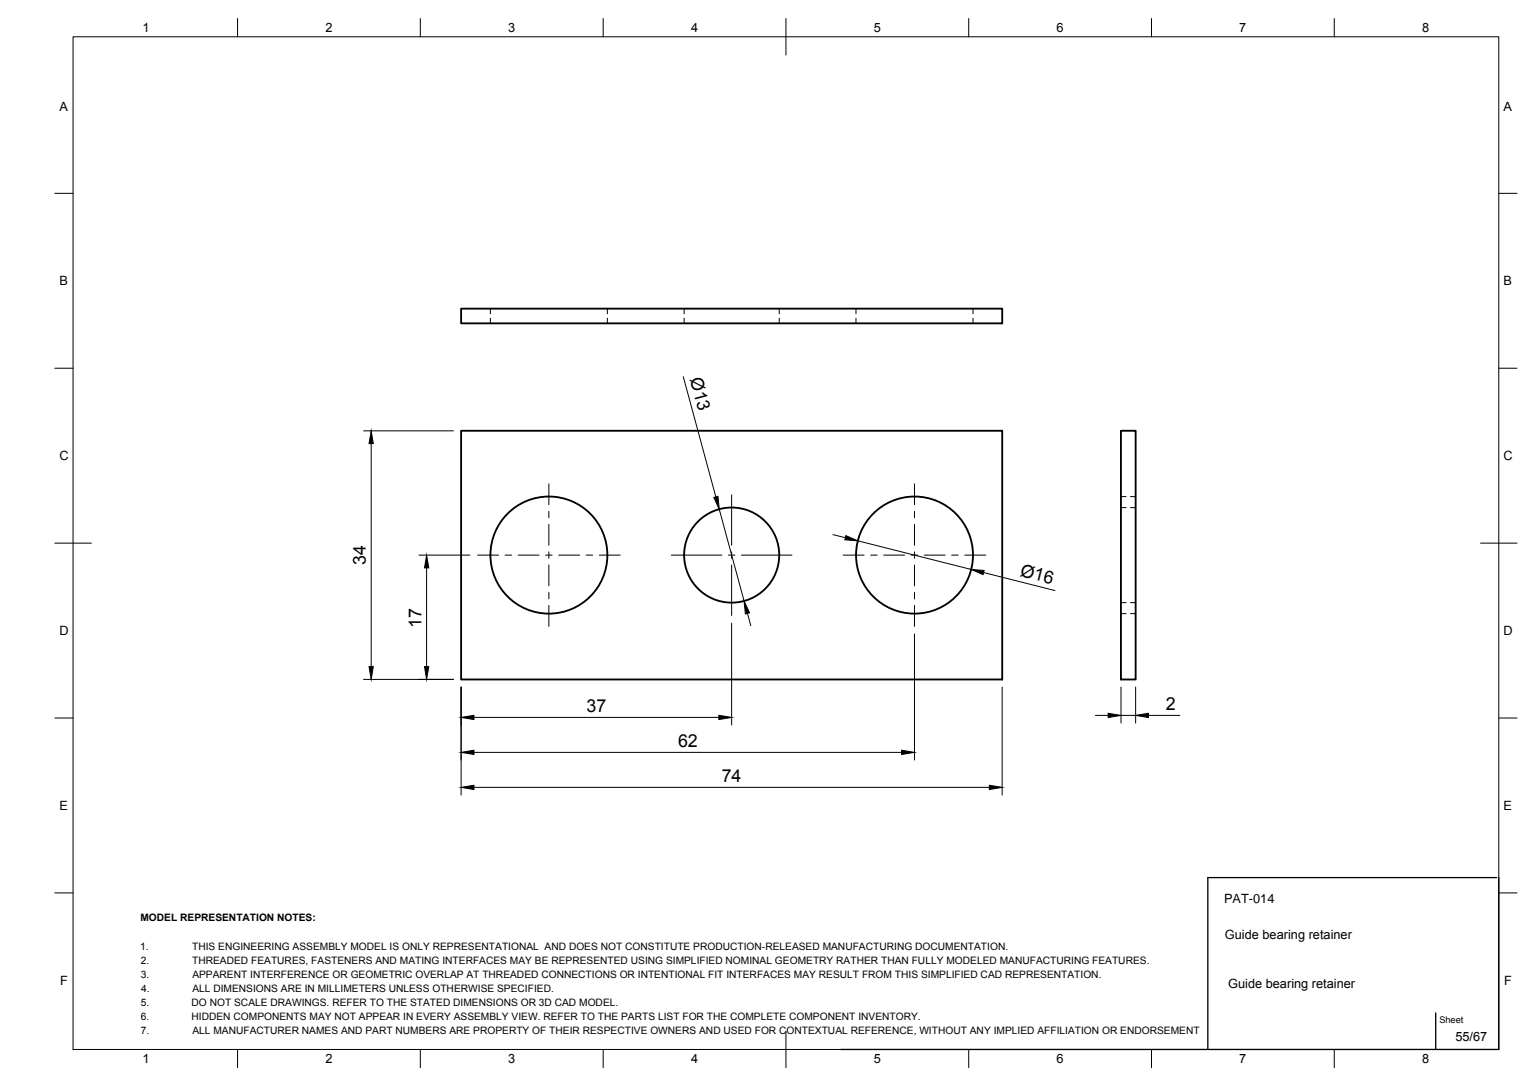
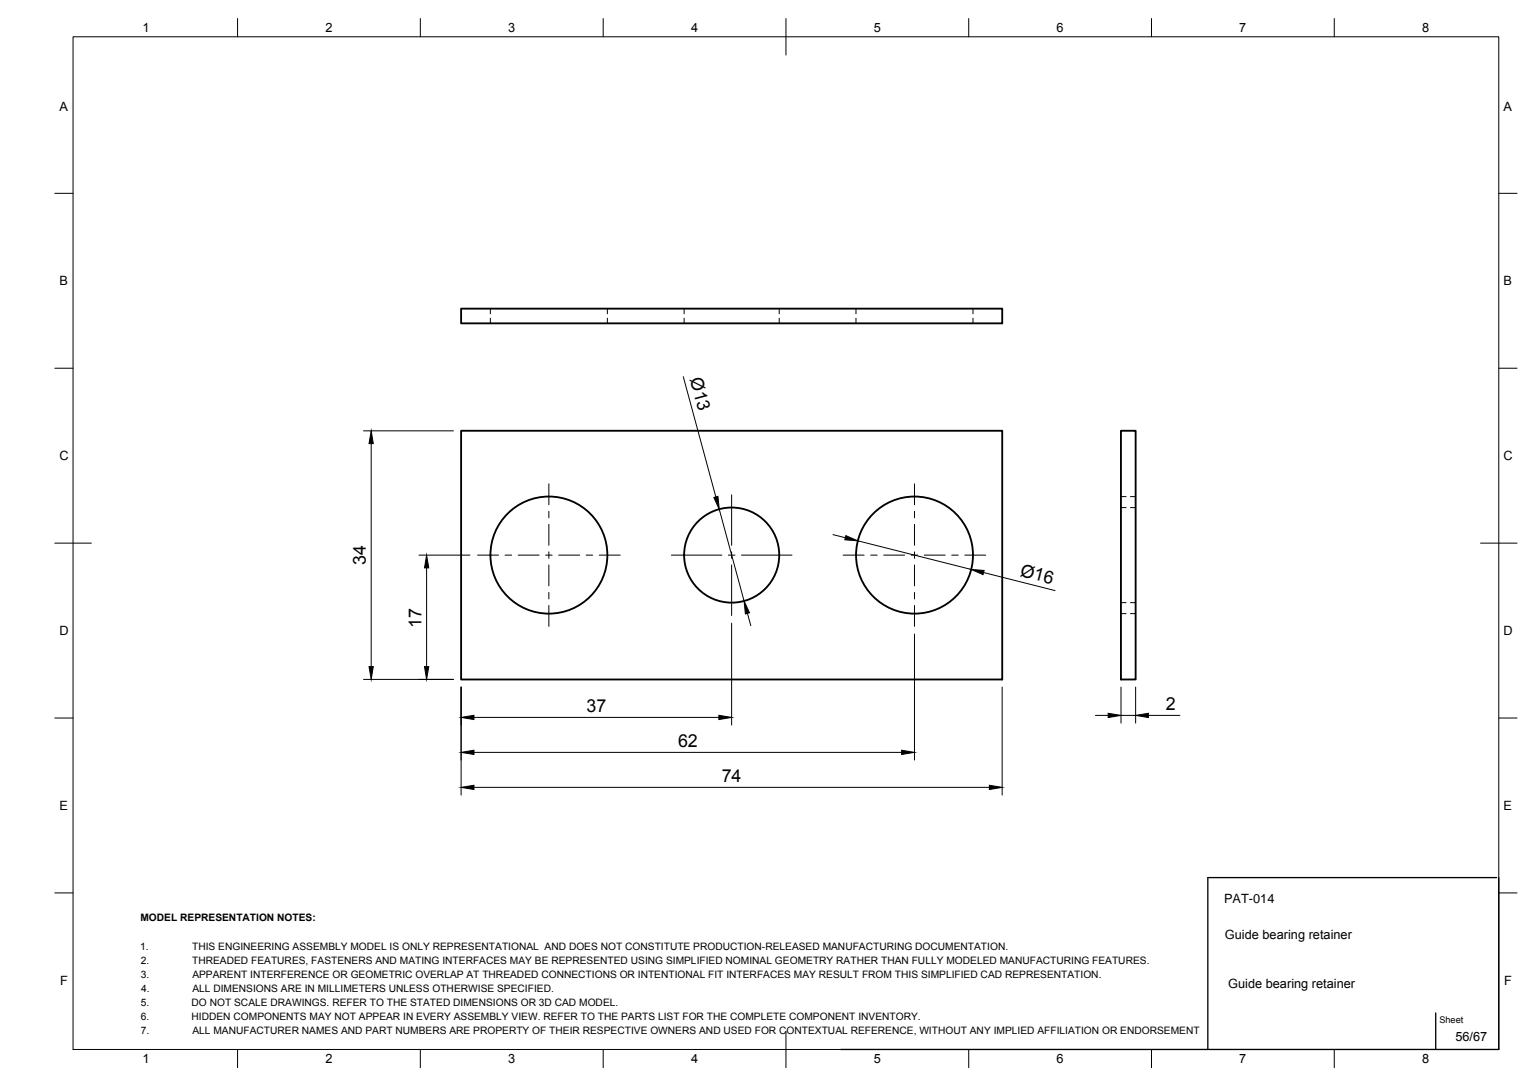
ISO-10303-21;
HEADER;
/* Generated by software containing ST-Developer
 * from STEP Tools, Inc. (www.steptools.com) 
 */

FILE_DESCRIPTION(
/* description */ ('Bin tilter linkage'),
/* implementation_level */ '2;1');

FILE_NAME(
/* name */ 'Guide bearing retainer.step',
/* time_stamp */ '2026-10-28T03:26:24-07:00',
/* author */ (''),
/* organization */ (''),
/* preprocessor_version */ 'ST-DEVELOPER v20.2',
/* originating_system */ 'Autodesk Translation Framework v15.17.0.0',
/* authorisation */ '');

FILE_SCHEMA (('AUTOMOTIVE_DESIGN { 1 0 10303 214 3 1 1 }'));
ENDSEC;

DATA;
#10=MECHANICAL_DESIGN_GEOMETRIC_PRESENTATION_REPRESENTATION('',(#961),#23728);
#741=SHAPE_REPRESENTATION_RELATIONSHIP('SRR','None',#24210,#847);
#847=ADVANCED_BREP_SHAPE_REPRESENTATION('',(#1073),#23710);
#961=STYLED_ITEM('',(#24765),#1073);
#1073=MANIFOLD_SOLID_BREP('Body1',#12493);
#1450=FACE_BOUND('',#3708,.T.);
#1451=FACE_BOUND('',#3709,.T.);
#1452=FACE_BOUND('',#3710,.T.);
#1453=FACE_BOUND('',#3712,.T.);
#1454=FACE_BOUND('',#3713,.T.);
#1455=FACE_BOUND('',#3714,.T.);
#1822=PLANE('',#15253);
#1823=PLANE('',#15254);
#1824=PLANE('',#15255);
#1825=PLANE('',#15256);
#1826=PLANE('',#15257);
#1827=PLANE('',#15258);
#2560=FACE_OUTER_BOUND('',#3700,.T.);
#2561=FACE_OUTER_BOUND('',#3701,.T.);
#2562=FACE_OUTER_BOUND('',#3702,.T.);
#2563=FACE_OUTER_BOUND('',#3703,.T.);
#2564=FACE_OUTER_BOUND('',#3704,.T.);
#2565=FACE_OUTER_BOUND('',#3705,.T.);
#2566=FACE_OUTER_BOUND('',#3706,.T.);
#2567=FACE_OUTER_BOUND('',#3707,.T.);
#2568=FACE_OUTER_BOUND('',#3711,.T.);
#3700=EDGE_LOOP('',(#10871,#10872,#10873,#10874));
#3701=EDGE_LOOP('',(#10875,#10876,#10877,#10878));
#3702=EDGE_LOOP('',(#10879,#10880,#10881,#10882));
#3703=EDGE_LOOP('',(#10883,#10884,#10885,#10886));
#3704=EDGE_LOOP('',(#10887,#10888,#10889,#10890));
#3705=EDGE_LOOP('',(#10891,#10892,#10893,#10894));
#3706=EDGE_LOOP('',(#10895,#10896,#10897,#10898));
#3707=EDGE_LOOP('',(#10899,#10900,#10901,#10902));
#3708=EDGE_LOOP('',(#10903));
#3709=EDGE_LOOP('',(#10904));
#3710=EDGE_LOOP('',(#10905));
#3711=EDGE_LOOP('',(#10906,#10907,#10908,#10909));
#3712=EDGE_LOOP('',(#10910));
#3713=EDGE_LOOP('',(#10911));
#3714=EDGE_LOOP('',(#10912));
#4407=LINE('',#23021,#5082);
#4408=LINE('',#23027,#5083);
#4409=LINE('',#23033,#5084);
#4410=LINE('',#23038,#5085);
#4411=LINE('',#23040,#5086);
#4412=LINE('',#23042,#5087);
#4413=LINE('',#23043,#5088);
#4414=LINE('',#23046,#5089);
#4415=LINE('',#23048,#5090);
#4416=LINE('',#23049,#5091);
#4417=LINE('',#23052,#5092);
#4418=LINE('',#23054,#5093);
#4419=LINE('',#23055,#5094);
#4420=LINE('',#23057,#5095);
#4421=LINE('',#23058,#5096);
#5082=VECTOR('',#19172,0.65);
#5083=VECTOR('',#19179,0.8);
#5084=VECTOR('',#19186,0.8);
#5085=VECTOR('',#19191,1.);
#5086=VECTOR('',#19192,1.);
#5087=VECTOR('',#19193,1.);
#5088=VECTOR('',#19194,1.);
#5089=VECTOR('',#19197,1.);
#5090=VECTOR('',#19198,1.);
#5091=VECTOR('',#19199,1.);
#5092=VECTOR('',#19202,1.);
#5093=VECTOR('',#19203,1.);
#5094=VECTOR('',#19204,1.);
#5095=VECTOR('',#19207,1.);
#5096=VECTOR('',#19208,1.);
#5876=CIRCLE('',#15245,0.65);
#5877=CIRCLE('',#15246,0.65);
#5878=CIRCLE('',#15248,0.8);
#5879=CIRCLE('',#15249,0.8);
#5880=CIRCLE('',#15251,0.8);
#5881=CIRCLE('',#15252,0.8);
#6795=VERTEX_POINT('',#23018);
#6796=VERTEX_POINT('',#23020);
#6797=VERTEX_POINT('',#23024);
#6798=VERTEX_POINT('',#23026);
#6799=VERTEX_POINT('',#23030);
#6800=VERTEX_POINT('',#23032);
#6801=VERTEX_POINT('',#23036);
#6802=VERTEX_POINT('',#23037);
#6803=VERTEX_POINT('',#23039);
#6804=VERTEX_POINT('',#23041);
#6805=VERTEX_POINT('',#23045);
#6806=VERTEX_POINT('',#23047);
#6807=VERTEX_POINT('',#23051);
#6808=VERTEX_POINT('',#23053);
#8175=EDGE_CURVE('',#6795,#6795,#5876,.T.);
#8176=EDGE_CURVE('',#6795,#6796,#4407,.T.);
#8177=EDGE_CURVE('',#6796,#6796,#5877,.T.);
#8178=EDGE_CURVE('',#6797,#6797,#5878,.T.);
#8179=EDGE_CURVE('',#6797,#6798,#4408,.T.);
#8180=EDGE_CURVE('',#6798,#6798,#5879,.T.);
#8181=EDGE_CURVE('',#6799,#6799,#5880,.T.);
#8182=EDGE_CURVE('',#6799,#6800,#4409,.T.);
#8183=EDGE_CURVE('',#6800,#6800,#5881,.T.);
#8184=EDGE_CURVE('',#6801,#6802,#4410,.T.);
#8185=EDGE_CURVE('',#6802,#6803,#4411,.T.);
#8186=EDGE_CURVE('',#6804,#6803,#4412,.T.);
#8187=EDGE_CURVE('',#6801,#6804,#4413,.T.);
#8188=EDGE_CURVE('',#6805,#6801,#4414,.T.);
#8189=EDGE_CURVE('',#6806,#6804,#4415,.T.);
#8190=EDGE_CURVE('',#6805,#6806,#4416,.T.);
#8191=EDGE_CURVE('',#6807,#6805,#4417,.T.);
#8192=EDGE_CURVE('',#6808,#6806,#4418,.T.);
#8193=EDGE_CURVE('',#6807,#6808,#4419,.T.);
#8194=EDGE_CURVE('',#6802,#6807,#4420,.T.);
#8195=EDGE_CURVE('',#6803,#6808,#4421,.T.);
#10871=ORIENTED_EDGE('',*,*,#8175,.F.);
#10872=ORIENTED_EDGE('',*,*,#8176,.T.);
#10873=ORIENTED_EDGE('',*,*,#8177,.F.);
#10874=ORIENTED_EDGE('',*,*,#8176,.F.);
#10875=ORIENTED_EDGE('',*,*,#8178,.F.);
#10876=ORIENTED_EDGE('',*,*,#8179,.T.);
#10877=ORIENTED_EDGE('',*,*,#8180,.F.);
#10878=ORIENTED_EDGE('',*,*,#8179,.F.);
#10879=ORIENTED_EDGE('',*,*,#8181,.F.);
#10880=ORIENTED_EDGE('',*,*,#8182,.T.);
#10881=ORIENTED_EDGE('',*,*,#8183,.F.);
#10882=ORIENTED_EDGE('',*,*,#8182,.F.);
#10883=ORIENTED_EDGE('',*,*,#8184,.T.);
#10884=ORIENTED_EDGE('',*,*,#8185,.T.);
#10885=ORIENTED_EDGE('',*,*,#8186,.F.);
#10886=ORIENTED_EDGE('',*,*,#8187,.F.);
#10887=ORIENTED_EDGE('',*,*,#8188,.T.);
#10888=ORIENTED_EDGE('',*,*,#8187,.T.);
#10889=ORIENTED_EDGE('',*,*,#8189,.F.);
#10890=ORIENTED_EDGE('',*,*,#8190,.F.);
#10891=ORIENTED_EDGE('',*,*,#8191,.T.);
#10892=ORIENTED_EDGE('',*,*,#8190,.T.);
#10893=ORIENTED_EDGE('',*,*,#8192,.F.);
#10894=ORIENTED_EDGE('',*,*,#8193,.F.);
#10895=ORIENTED_EDGE('',*,*,#8194,.T.);
#10896=ORIENTED_EDGE('',*,*,#8193,.T.);
#10897=ORIENTED_EDGE('',*,*,#8195,.F.);
#10898=ORIENTED_EDGE('',*,*,#8185,.F.);
#10899=ORIENTED_EDGE('',*,*,#8195,.T.);
#10900=ORIENTED_EDGE('',*,*,#8192,.T.);
#10901=ORIENTED_EDGE('',*,*,#8189,.T.);
#10902=ORIENTED_EDGE('',*,*,#8186,.T.);
#10903=ORIENTED_EDGE('',*,*,#8177,.T.);
#10904=ORIENTED_EDGE('',*,*,#8180,.T.);
#10905=ORIENTED_EDGE('',*,*,#8183,.T.);
#10906=ORIENTED_EDGE('',*,*,#8194,.F.);
#10907=ORIENTED_EDGE('',*,*,#8184,.F.);
#10908=ORIENTED_EDGE('',*,*,#8188,.F.);
#10909=ORIENTED_EDGE('',*,*,#8191,.F.);
#10910=ORIENTED_EDGE('',*,*,#8175,.T.);
#10911=ORIENTED_EDGE('',*,*,#8178,.T.);
#10912=ORIENTED_EDGE('',*,*,#8181,.T.);
#11579=CYLINDRICAL_SURFACE('',#15244,0.65);
#11580=CYLINDRICAL_SURFACE('',#15247,0.8);
#11581=CYLINDRICAL_SURFACE('',#15250,0.8);
#12285=ADVANCED_FACE('',(#2560),#11579,.F.);
#12286=ADVANCED_FACE('',(#2561),#11580,.F.);
#12287=ADVANCED_FACE('',(#2562),#11581,.F.);
#12288=ADVANCED_FACE('',(#2563),#1822,.T.);
#12289=ADVANCED_FACE('',(#2564),#1823,.T.);
#12290=ADVANCED_FACE('',(#2565),#1824,.T.);
#12291=ADVANCED_FACE('',(#2566),#1825,.T.);
#12292=ADVANCED_FACE('',(#2567,#1450,#1451,#1452),#1826,.T.);
#12293=ADVANCED_FACE('',(#2568,#1453,#1454,#1455),#1827,.F.);
#12493=CLOSED_SHELL('',(#12285,#12286,#12287,#12288,#12289,#12290,#12291,
#12292,#12293));
#15243=AXIS2_PLACEMENT_3D('',#23016,#19166,#19167);
#15244=AXIS2_PLACEMENT_3D('',#23017,#19168,#19169);
#15245=AXIS2_PLACEMENT_3D('',#23019,#19170,#19171);
#15246=AXIS2_PLACEMENT_3D('',#23022,#19173,#19174);
#15247=AXIS2_PLACEMENT_3D('',#23023,#19175,#19176);
#15248=AXIS2_PLACEMENT_3D('',#23025,#19177,#19178);
#15249=AXIS2_PLACEMENT_3D('',#23028,#19180,#19181);
#15250=AXIS2_PLACEMENT_3D('',#23029,#19182,#19183);
#15251=AXIS2_PLACEMENT_3D('',#23031,#19184,#19185);
#15252=AXIS2_PLACEMENT_3D('',#23034,#19187,#19188);
#15253=AXIS2_PLACEMENT_3D('',#23035,#19189,#19190);
#15254=AXIS2_PLACEMENT_3D('',#23044,#19195,#19196);
#15255=AXIS2_PLACEMENT_3D('',#23050,#19200,#19201);
#15256=AXIS2_PLACEMENT_3D('',#23056,#19205,#19206);
#15257=AXIS2_PLACEMENT_3D('',#23059,#19209,#19210);
#15258=AXIS2_PLACEMENT_3D('',#23060,#19211,#19212);
#19166=DIRECTION('axis',(0.,0.,1.));
#19167=DIRECTION('refdir',(1.,0.,0.));
#19168=DIRECTION('center_axis',(1.,0.,0.));
#19169=DIRECTION('ref_axis',(0.,0.,-1.));
#19170=DIRECTION('center_axis',(1.,0.,0.));
#19171=DIRECTION('ref_axis',(0.,0.,-1.));
#19172=DIRECTION('',(1.,0.,0.));
#19173=DIRECTION('center_axis',(-1.,0.,0.));
#19174=DIRECTION('ref_axis',(0.,0.,-1.));
#19175=DIRECTION('center_axis',(1.,0.,0.));
#19176=DIRECTION('ref_axis',(0.,0.,-1.));
#19177=DIRECTION('center_axis',(1.,0.,0.));
#19178=DIRECTION('ref_axis',(0.,0.,-1.));
#19179=DIRECTION('',(1.,0.,0.));
#19180=DIRECTION('center_axis',(-1.,0.,0.));
#19181=DIRECTION('ref_axis',(0.,0.,-1.));
#19182=DIRECTION('center_axis',(1.,0.,0.));
#19183=DIRECTION('ref_axis',(0.,0.,-1.));
#19184=DIRECTION('center_axis',(1.,0.,0.));
#19185=DIRECTION('ref_axis',(0.,0.,-1.));
#19186=DIRECTION('',(1.,0.,0.));
#19187=DIRECTION('center_axis',(-1.,0.,0.));
#19188=DIRECTION('ref_axis',(0.,0.,-1.));
#19189=DIRECTION('center_axis',(0.,0.,1.));
#19190=DIRECTION('ref_axis',(0.,-1.,0.));
#19191=DIRECTION('',(0.,-1.,0.));
#19192=DIRECTION('',(1.,0.,0.));
#19193=DIRECTION('',(0.,-1.,0.));
#19194=DIRECTION('',(1.,0.,0.));
#19195=DIRECTION('center_axis',(0.,1.,0.));
#19196=DIRECTION('ref_axis',(0.,0.,1.));
#19197=DIRECTION('',(0.,0.,1.));
#19198=DIRECTION('',(0.,0.,1.));
#19199=DIRECTION('',(1.,0.,0.));
#19200=DIRECTION('center_axis',(0.,0.,-1.));
#19201=DIRECTION('ref_axis',(0.,1.,0.));
#19202=DIRECTION('',(0.,1.,0.));
#19203=DIRECTION('',(0.,1.,0.));
#19204=DIRECTION('',(1.,0.,0.));
#19205=DIRECTION('center_axis',(0.,-1.,0.));
#19206=DIRECTION('ref_axis',(0.,0.,-1.));
#19207=DIRECTION('',(0.,0.,-1.));
#19208=DIRECTION('',(0.,0.,-1.));
#19209=DIRECTION('center_axis',(1.,0.,0.));
#19210=DIRECTION('ref_axis',(0.,0.,-1.));
#19211=DIRECTION('center_axis',(1.,0.,0.));
#19212=DIRECTION('ref_axis',(0.,0.,-1.));
#23016=CARTESIAN_POINT('',(0.,0.,0.));
#23017=CARTESIAN_POINT('Origin',(-6.,-4.5,8.));
#23018=CARTESIAN_POINT('',(-5.9,-4.5,8.65));
#23019=CARTESIAN_POINT('Origin',(-5.9,-4.5,8.));
#23020=CARTESIAN_POINT('',(-5.7,-4.5,8.65));
#23021=CARTESIAN_POINT('',(-6.,-4.5,8.65));
#23022=CARTESIAN_POINT('Origin',(-5.7,-4.5,8.));
#23023=CARTESIAN_POINT('Origin',(-6.,-7.,8.));
#23024=CARTESIAN_POINT('',(-5.9,-7.,8.8));
#23025=CARTESIAN_POINT('Origin',(-5.9,-7.,8.));
#23026=CARTESIAN_POINT('',(-5.7,-7.,8.8));
#23027=CARTESIAN_POINT('',(-6.,-7.,8.8));
#23028=CARTESIAN_POINT('Origin',(-5.7,-7.,8.));
#23029=CARTESIAN_POINT('Origin',(-6.,-2.,8.));
#23030=CARTESIAN_POINT('',(-5.9,-2.,8.8));
#23031=CARTESIAN_POINT('Origin',(-5.9,-2.,8.));
#23032=CARTESIAN_POINT('',(-5.7,-2.,8.8));
#23033=CARTESIAN_POINT('',(-6.,-2.,8.8));
#23034=CARTESIAN_POINT('Origin',(-5.7,-2.,8.));
#23035=CARTESIAN_POINT('Origin',(-5.9,-0.8,9.7));
#23036=CARTESIAN_POINT('',(-5.9,-0.8,9.7));
#23037=CARTESIAN_POINT('',(-5.9,-8.2,9.7));
#23038=CARTESIAN_POINT('',(-5.9,-0.8,9.7));
#23039=CARTESIAN_POINT('',(-5.7,-8.2,9.7));
#23040=CARTESIAN_POINT('',(-5.9,-8.2,9.7));
#23041=CARTESIAN_POINT('',(-5.7,-0.8,9.7));
#23042=CARTESIAN_POINT('',(-5.7,-0.8,9.7));
#23043=CARTESIAN_POINT('',(-5.9,-0.8,9.7));
#23044=CARTESIAN_POINT('Origin',(-5.9,-0.8,6.3));
#23045=CARTESIAN_POINT('',(-5.9,-0.8,6.3));
#23046=CARTESIAN_POINT('',(-5.9,-0.8,6.3));
#23047=CARTESIAN_POINT('',(-5.7,-0.8,6.3));
#23048=CARTESIAN_POINT('',(-5.7,-0.8,6.3));
#23049=CARTESIAN_POINT('',(-5.9,-0.8,6.3));
#23050=CARTESIAN_POINT('Origin',(-5.9,-8.2,6.3));
#23051=CARTESIAN_POINT('',(-5.9,-8.2,6.3));
#23052=CARTESIAN_POINT('',(-5.9,-8.2,6.3));
#23053=CARTESIAN_POINT('',(-5.7,-8.2,6.3));
#23054=CARTESIAN_POINT('',(-5.7,-8.2,6.3));
#23055=CARTESIAN_POINT('',(-5.9,-8.2,6.3));
#23056=CARTESIAN_POINT('Origin',(-5.9,-8.2,9.7));
#23057=CARTESIAN_POINT('',(-5.9,-8.2,9.7));
#23058=CARTESIAN_POINT('',(-5.7,-8.2,9.7));
#23059=CARTESIAN_POINT('Origin',(-5.7,-4.5,8.));
#23060=CARTESIAN_POINT('Origin',(-5.9,-4.5,8.));
#23593=UNCERTAINTY_MEASURE_WITH_UNIT(LENGTH_MEASURE(0.001),#23729,
'DISTANCE_ACCURACY_VALUE',
'Maximum model space distance between geometric entities at asserted c
onnectivities');
#23611=UNCERTAINTY_MEASURE_WITH_UNIT(LENGTH_MEASURE(0.001),#23729,
'DISTANCE_ACCURACY_VALUE',
'Maximum model space distance between geometric entities at asserted c
onnectivities');
#23710=(
GEOMETRIC_REPRESENTATION_CONTEXT(3)
GLOBAL_UNCERTAINTY_ASSIGNED_CONTEXT((#23593))
GLOBAL_UNIT_ASSIGNED_CONTEXT((#23729,#23731,#23732))
REPRESENTATION_CONTEXT('','3D')
);
#23728=(
GEOMETRIC_REPRESENTATION_CONTEXT(3)
GLOBAL_UNCERTAINTY_ASSIGNED_CONTEXT((#23611))
GLOBAL_UNIT_ASSIGNED_CONTEXT((#23729,#23731,#23732))
REPRESENTATION_CONTEXT('','3D')
);
#23729=(
LENGTH_UNIT()
NAMED_UNIT(*)
SI_UNIT(.CENTI.,.METRE.)
);
#23731=(
NAMED_UNIT(*)
PLANE_ANGLE_UNIT()
SI_UNIT($,.RADIAN.)
);
#23732=(
NAMED_UNIT(*)
SI_UNIT($,.STERADIAN.)
SOLID_ANGLE_UNIT()
);
#23831=SHAPE_DEFINITION_REPRESENTATION(#24069,#24210);
#24069=PRODUCT_DEFINITION_SHAPE('',$,#24327);
#24210=SHAPE_REPRESENTATION('',(#15243),#23710);
#24228=PRODUCT_DEFINITION_CONTEXT('part definition',#24578,'design');
#24327=PRODUCT_DEFINITION('Guide bearing retainer',
'Guide bearing retainer',#24443,#24228);
#24443=PRODUCT_DEFINITION_FORMATION('',$,#24678);
#24578=APPLICATION_CONTEXT(
'Core Data for Automotive Mechanical Design Process');
#24579=PRODUCT_CONTEXT('part definition',#24578,'mechanical');
#24678=PRODUCT('Guide bearing retainer','Guide bearing retainer',
'Guide bearing retainer',(#24579));
#24759=COLOUR_RGB('Grey',0.48,0.52,0.57);
#24760=FILL_AREA_STYLE_COLOUR('',#24759);
#24761=FILL_AREA_STYLE('',(#24760));
#24762=SURFACE_STYLE_FILL_AREA(#24761);
#24763=SURFACE_SIDE_STYLE('',(#24762));
#24764=SURFACE_STYLE_USAGE(.BOTH.,#24763);
#24765=PRESENTATION_STYLE_ASSIGNMENT((#24764));
ENDSEC;
END-ISO-10303-21;
